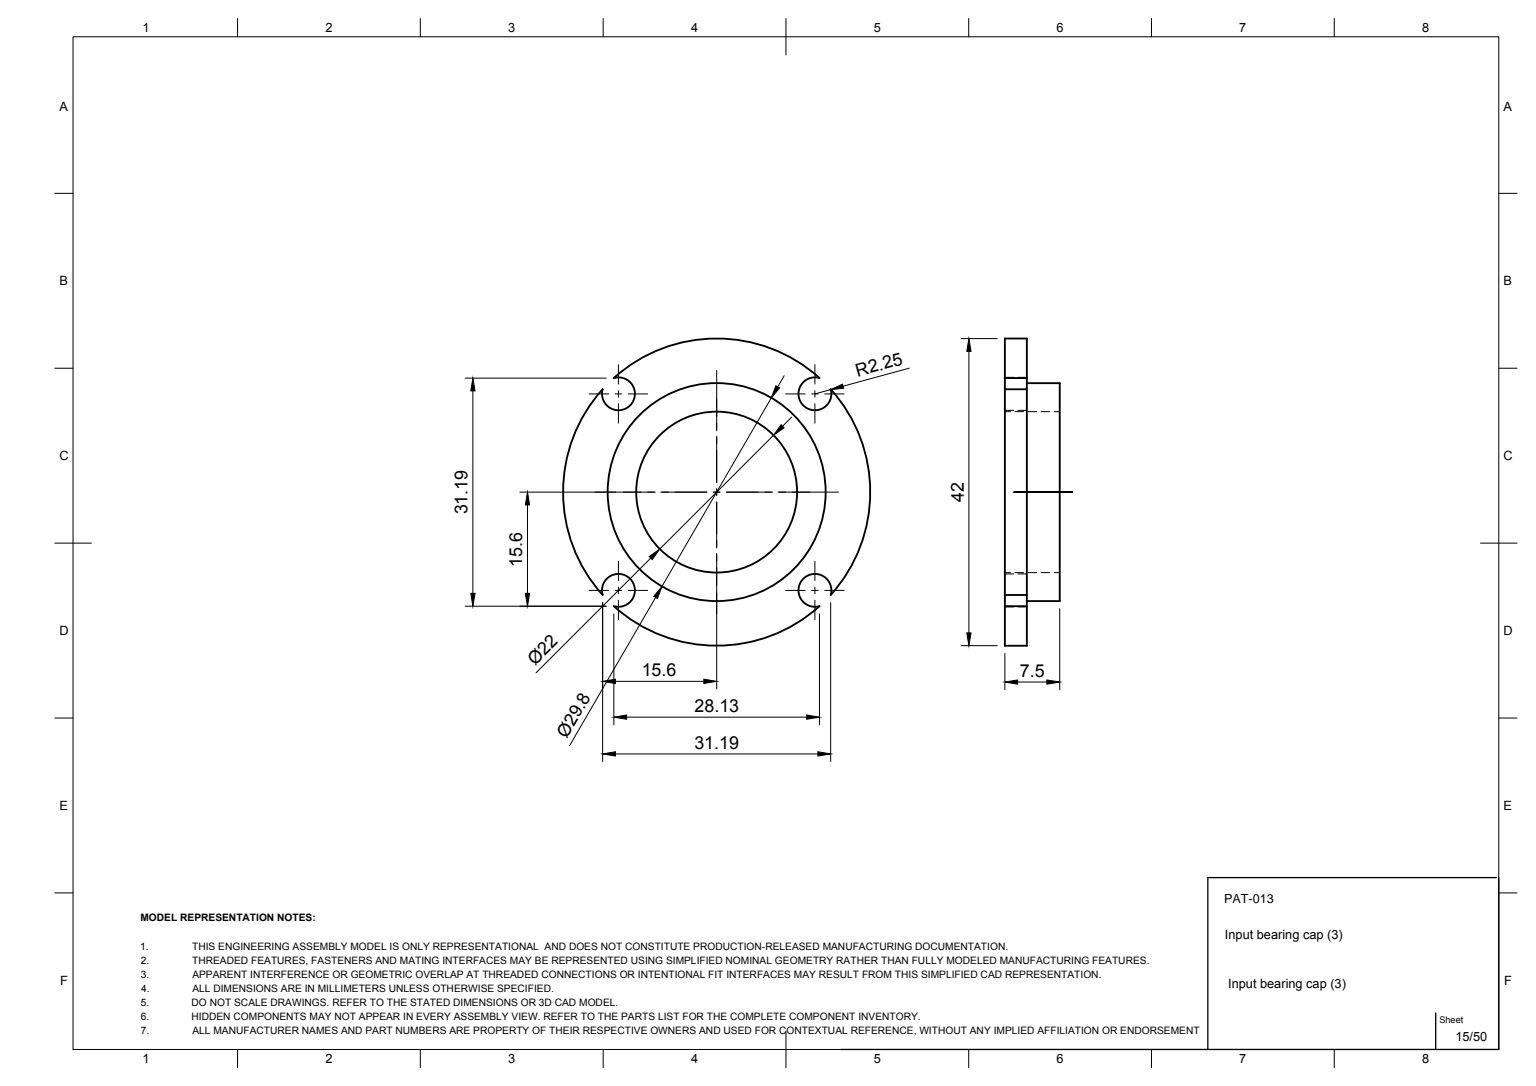
ISO-10303-21;
HEADER;
/* Generated by software containing ST-Developer
 * from STEP Tools, Inc. (www.steptools.com) 
 */

FILE_DESCRIPTION(
/* description */ ('Belt-driven linear axis on 2020 extrusion'),
/* implementation_level */ '2;1');

FILE_NAME(
/* name */ 'Input bearing cap (3).step',
/* time_stamp */ '2026-10-28T03:26:09-07:00',
/* author */ (''),
/* organization */ (''),
/* preprocessor_version */ 'ST-DEVELOPER v20.2',
/* originating_system */ 'Autodesk Translation Framework v15.17.0.0',
/* authorisation */ '');

FILE_SCHEMA (('AUTOMOTIVE_DESIGN { 1 0 10303 214 3 1 1 }'));
ENDSEC;

DATA;
#10=MECHANICAL_DESIGN_GEOMETRIC_PRESENTATION_REPRESENTATION('',(#622),#20096);
#528=SHAPE_REPRESENTATION_RELATIONSHIP('SRR','None',#20324,#574);
#574=ADVANCED_BREP_SHAPE_REPRESENTATION('',(#678),#20055);
#622=STYLED_ITEM('',(#20650),#678);
#678=MANIFOLD_SOLID_BREP('Body1',#10935);
#791=FACE_BOUND('',#2101,.T.);
#792=FACE_BOUND('',#2108,.T.);
#793=FACE_BOUND('',#2111,.T.);
#968=PLANE('',#11810);
#969=PLANE('',#11826);
#970=PLANE('',#11830);
#1401=FACE_OUTER_BOUND('',#2096,.T.);
#1402=FACE_OUTER_BOUND('',#2097,.T.);
#1403=FACE_OUTER_BOUND('',#2098,.T.);
#1404=FACE_OUTER_BOUND('',#2099,.T.);
#1405=FACE_OUTER_BOUND('',#2100,.T.);
#1406=FACE_OUTER_BOUND('',#2102,.T.);
#1407=FACE_OUTER_BOUND('',#2103,.T.);
#1408=FACE_OUTER_BOUND('',#2104,.T.);
#1409=FACE_OUTER_BOUND('',#2105,.T.);
#1410=FACE_OUTER_BOUND('',#2106,.T.);
#1411=FACE_OUTER_BOUND('',#2107,.T.);
#1412=FACE_OUTER_BOUND('',#2109,.T.);
#1413=FACE_OUTER_BOUND('',#2110,.T.);
#2096=EDGE_LOOP('',(#7901,#7902,#7903,#7904));
#2097=EDGE_LOOP('',(#7905,#7906,#7907,#7908));
#2098=EDGE_LOOP('',(#7909,#7910,#7911,#7912));
#2099=EDGE_LOOP('',(#7913,#7914,#7915,#7916));
#2100=EDGE_LOOP('',(#7917,#7918,#7919,#7920,#7921,#7922,#7923,#7924));
#2101=EDGE_LOOP('',(#7925));
#2102=EDGE_LOOP('',(#7926,#7927,#7928,#7929));
#2103=EDGE_LOOP('',(#7930,#7931,#7932,#7933));
#2104=EDGE_LOOP('',(#7934,#7935,#7936,#7937));
#2105=EDGE_LOOP('',(#7938,#7939,#7940,#7941));
#2106=EDGE_LOOP('',(#7942,#7943,#7944,#7945));
#2107=EDGE_LOOP('',(#7946));
#2108=EDGE_LOOP('',(#7947));
#2109=EDGE_LOOP('',(#7948,#7949,#7950,#7951));
#2110=EDGE_LOOP('',(#7952,#7953,#7954,#7955,#7956,#7957,#7958,#7959));
#2111=EDGE_LOOP('',(#7960));
#2845=LINE('',#16939,#3702);
#2846=LINE('',#16943,#3703);
#2847=LINE('',#16948,#3704);
#2848=LINE('',#16952,#3705);
#2849=LINE('',#16957,#3706);
#2850=LINE('',#16961,#3707);
#2851=LINE('',#16966,#3708);
#2852=LINE('',#16970,#3709);
#2853=LINE('',#16989,#3710);
#2854=LINE('',#16997,#3711);
#3702=VECTOR('',#13583,1.);
#3703=VECTOR('',#13586,1.);
#3704=VECTOR('',#13591,1.);
#3705=VECTOR('',#13594,1.);
#3706=VECTOR('',#13599,1.);
#3707=VECTOR('',#13602,1.);
#3708=VECTOR('',#13607,1.);
#3709=VECTOR('',#13610,1.);
#3710=VECTOR('',#13643,1.49);
#3711=VECTOR('',#13654,1.1);
#4523=CIRCLE('',#11799,0.225000000000001);
#4524=CIRCLE('',#11800,0.225000000000001);
#4525=CIRCLE('',#11802,0.225000000000001);
#4526=CIRCLE('',#11803,0.225000000000001);
#4527=CIRCLE('',#11805,0.225000000000001);
#4528=CIRCLE('',#11806,0.225000000000001);
#4529=CIRCLE('',#11808,0.225000000000001);
#4530=CIRCLE('',#11809,0.225000000000001);
#4531=CIRCLE('',#11811,2.1);
#4532=CIRCLE('',#11812,2.1);
#4533=CIRCLE('',#11813,2.1);
#4534=CIRCLE('',#11814,2.1);
#4535=CIRCLE('',#11815,1.49);
#4536=CIRCLE('',#11817,2.1);
#4537=CIRCLE('',#11819,2.1);
#4538=CIRCLE('',#11821,2.1);
#4539=CIRCLE('',#11823,2.1);
#4540=CIRCLE('',#11825,1.49);
#4541=CIRCLE('',#11827,1.1);
#4542=CIRCLE('',#11829,1.1);
#5108=VERTEX_POINT('',#16937);
#5109=VERTEX_POINT('',#16938);
#5110=VERTEX_POINT('',#16940);
#5111=VERTEX_POINT('',#16942);
#5112=VERTEX_POINT('',#16946);
#5113=VERTEX_POINT('',#16947);
#5114=VERTEX_POINT('',#16949);
#5115=VERTEX_POINT('',#16951);
#5116=VERTEX_POINT('',#16955);
#5117=VERTEX_POINT('',#16956);
#5118=VERTEX_POINT('',#16958);
#5119=VERTEX_POINT('',#16960);
#5120=VERTEX_POINT('',#16964);
#5121=VERTEX_POINT('',#16965);
#5122=VERTEX_POINT('',#16967);
#5123=VERTEX_POINT('',#16969);
#5124=VERTEX_POINT('',#16977);
#5125=VERTEX_POINT('',#16988);
#5126=VERTEX_POINT('',#16992);
#5127=VERTEX_POINT('',#16995);
#6165=EDGE_CURVE('',#5108,#5109,#2845,.T.);
#6166=EDGE_CURVE('',#5110,#5108,#4523,.T.);
#6167=EDGE_CURVE('',#5111,#5110,#2846,.T.);
#6168=EDGE_CURVE('',#5109,#5111,#4524,.T.);
#6169=EDGE_CURVE('',#5112,#5113,#2847,.T.);
#6170=EDGE_CURVE('',#5114,#5112,#4525,.T.);
#6171=EDGE_CURVE('',#5115,#5114,#2848,.T.);
#6172=EDGE_CURVE('',#5113,#5115,#4526,.T.);
#6173=EDGE_CURVE('',#5116,#5117,#2849,.T.);
#6174=EDGE_CURVE('',#5118,#5116,#4527,.T.);
#6175=EDGE_CURVE('',#5119,#5118,#2850,.T.);
#6176=EDGE_CURVE('',#5117,#5119,#4528,.T.);
#6177=EDGE_CURVE('',#5120,#5121,#2851,.T.);
#6178=EDGE_CURVE('',#5122,#5120,#4529,.T.);
#6179=EDGE_CURVE('',#5123,#5122,#2852,.T.);
#6180=EDGE_CURVE('',#5121,#5123,#4530,.T.);
#6181=EDGE_CURVE('',#5122,#5108,#4531,.T.);
#6182=EDGE_CURVE('',#5118,#5120,#4532,.T.);
#6183=EDGE_CURVE('',#5114,#5116,#4533,.T.);
#6184=EDGE_CURVE('',#5110,#5112,#4534,.T.);
#6185=EDGE_CURVE('',#5124,#5124,#4535,.T.);
#6186=EDGE_CURVE('',#5119,#5121,#4536,.T.);
#6187=EDGE_CURVE('',#5115,#5117,#4537,.T.);
#6188=EDGE_CURVE('',#5123,#5109,#4538,.T.);
#6189=EDGE_CURVE('',#5111,#5113,#4539,.T.);
#6190=EDGE_CURVE('',#5124,#5125,#2853,.T.);
#6191=EDGE_CURVE('',#5125,#5125,#4540,.T.);
#6192=EDGE_CURVE('',#5126,#5126,#4541,.T.);
#6193=EDGE_CURVE('',#5127,#5127,#4542,.T.);
#6194=EDGE_CURVE('',#5127,#5126,#2854,.T.);
#7901=ORIENTED_EDGE('',*,*,#6165,.F.);
#7902=ORIENTED_EDGE('',*,*,#6166,.F.);
#7903=ORIENTED_EDGE('',*,*,#6167,.F.);
#7904=ORIENTED_EDGE('',*,*,#6168,.F.);
#7905=ORIENTED_EDGE('',*,*,#6169,.F.);
#7906=ORIENTED_EDGE('',*,*,#6170,.F.);
#7907=ORIENTED_EDGE('',*,*,#6171,.F.);
#7908=ORIENTED_EDGE('',*,*,#6172,.F.);
#7909=ORIENTED_EDGE('',*,*,#6173,.F.);
#7910=ORIENTED_EDGE('',*,*,#6174,.F.);
#7911=ORIENTED_EDGE('',*,*,#6175,.F.);
#7912=ORIENTED_EDGE('',*,*,#6176,.F.);
#7913=ORIENTED_EDGE('',*,*,#6177,.F.);
#7914=ORIENTED_EDGE('',*,*,#6178,.F.);
#7915=ORIENTED_EDGE('',*,*,#6179,.F.);
#7916=ORIENTED_EDGE('',*,*,#6180,.F.);
#7917=ORIENTED_EDGE('',*,*,#6166,.T.);
#7918=ORIENTED_EDGE('',*,*,#6181,.F.);
#7919=ORIENTED_EDGE('',*,*,#6178,.T.);
#7920=ORIENTED_EDGE('',*,*,#6182,.F.);
#7921=ORIENTED_EDGE('',*,*,#6174,.T.);
#7922=ORIENTED_EDGE('',*,*,#6183,.F.);
#7923=ORIENTED_EDGE('',*,*,#6170,.T.);
#7924=ORIENTED_EDGE('',*,*,#6184,.F.);
#7925=ORIENTED_EDGE('',*,*,#6185,.T.);
#7926=ORIENTED_EDGE('',*,*,#6175,.T.);
#7927=ORIENTED_EDGE('',*,*,#6182,.T.);
#7928=ORIENTED_EDGE('',*,*,#6177,.T.);
#7929=ORIENTED_EDGE('',*,*,#6186,.F.);
#7930=ORIENTED_EDGE('',*,*,#6171,.T.);
#7931=ORIENTED_EDGE('',*,*,#6183,.T.);
#7932=ORIENTED_EDGE('',*,*,#6173,.T.);
#7933=ORIENTED_EDGE('',*,*,#6187,.F.);
#7934=ORIENTED_EDGE('',*,*,#6165,.T.);
#7935=ORIENTED_EDGE('',*,*,#6188,.F.);
#7936=ORIENTED_EDGE('',*,*,#6179,.T.);
#7937=ORIENTED_EDGE('',*,*,#6181,.T.);
#7938=ORIENTED_EDGE('',*,*,#6167,.T.);
#7939=ORIENTED_EDGE('',*,*,#6184,.T.);
#7940=ORIENTED_EDGE('',*,*,#6169,.T.);
#7941=ORIENTED_EDGE('',*,*,#6189,.F.);
#7942=ORIENTED_EDGE('',*,*,#6185,.F.);
#7943=ORIENTED_EDGE('',*,*,#6190,.T.);
#7944=ORIENTED_EDGE('',*,*,#6191,.T.);
#7945=ORIENTED_EDGE('',*,*,#6190,.F.);
#7946=ORIENTED_EDGE('',*,*,#6191,.F.);
#7947=ORIENTED_EDGE('',*,*,#6192,.F.);
#7948=ORIENTED_EDGE('',*,*,#6193,.F.);
#7949=ORIENTED_EDGE('',*,*,#6194,.T.);
#7950=ORIENTED_EDGE('',*,*,#6192,.T.);
#7951=ORIENTED_EDGE('',*,*,#6194,.F.);
#7952=ORIENTED_EDGE('',*,*,#6168,.T.);
#7953=ORIENTED_EDGE('',*,*,#6189,.T.);
#7954=ORIENTED_EDGE('',*,*,#6172,.T.);
#7955=ORIENTED_EDGE('',*,*,#6187,.T.);
#7956=ORIENTED_EDGE('',*,*,#6176,.T.);
#7957=ORIENTED_EDGE('',*,*,#6186,.T.);
#7958=ORIENTED_EDGE('',*,*,#6180,.T.);
#7959=ORIENTED_EDGE('',*,*,#6188,.T.);
#7960=ORIENTED_EDGE('',*,*,#6193,.T.);
#10149=CYLINDRICAL_SURFACE('',#11798,0.225000000000001);
#10150=CYLINDRICAL_SURFACE('',#11801,0.225000000000001);
#10151=CYLINDRICAL_SURFACE('',#11804,0.225000000000001);
#10152=CYLINDRICAL_SURFACE('',#11807,0.225000000000001);
#10153=CYLINDRICAL_SURFACE('',#11816,2.1);
#10154=CYLINDRICAL_SURFACE('',#11818,2.1);
#10155=CYLINDRICAL_SURFACE('',#11820,2.1);
#10156=CYLINDRICAL_SURFACE('',#11822,2.1);
#10157=CYLINDRICAL_SURFACE('',#11824,1.49);
#10158=CYLINDRICAL_SURFACE('',#11828,1.1);
#10452=ADVANCED_FACE('',(#1401),#10149,.F.);
#10453=ADVANCED_FACE('',(#1402),#10150,.F.);
#10454=ADVANCED_FACE('',(#1403),#10151,.F.);
#10455=ADVANCED_FACE('',(#1404),#10152,.F.);
#10456=ADVANCED_FACE('',(#1405,#791),#968,.F.);
#10457=ADVANCED_FACE('',(#1406),#10153,.T.);
#10458=ADVANCED_FACE('',(#1407),#10154,.T.);
#10459=ADVANCED_FACE('',(#1408),#10155,.T.);
#10460=ADVANCED_FACE('',(#1409),#10156,.T.);
#10461=ADVANCED_FACE('',(#1410),#10157,.T.);
#10462=ADVANCED_FACE('',(#1411,#792),#969,.F.);
#10463=ADVANCED_FACE('',(#1412),#10158,.F.);
#10464=ADVANCED_FACE('',(#1413,#793),#970,.T.);
#10935=CLOSED_SHELL('',(#10452,#10453,#10454,#10455,#10456,#10457,#10458,
#10459,#10460,#10461,#10462,#10463,#10464));
#11797=AXIS2_PLACEMENT_3D('',#16935,#13579,#13580);
#11798=AXIS2_PLACEMENT_3D('',#16936,#13581,#13582);
#11799=AXIS2_PLACEMENT_3D('',#16941,#13584,#13585);
#11800=AXIS2_PLACEMENT_3D('',#16944,#13587,#13588);
#11801=AXIS2_PLACEMENT_3D('',#16945,#13589,#13590);
#11802=AXIS2_PLACEMENT_3D('',#16950,#13592,#13593);
#11803=AXIS2_PLACEMENT_3D('',#16953,#13595,#13596);
#11804=AXIS2_PLACEMENT_3D('',#16954,#13597,#13598);
#11805=AXIS2_PLACEMENT_3D('',#16959,#13600,#13601);
#11806=AXIS2_PLACEMENT_3D('',#16962,#13603,#13604);
#11807=AXIS2_PLACEMENT_3D('',#16963,#13605,#13606);
#11808=AXIS2_PLACEMENT_3D('',#16968,#13608,#13609);
#11809=AXIS2_PLACEMENT_3D('',#16971,#13611,#13612);
#11810=AXIS2_PLACEMENT_3D('',#16972,#13613,#13614);
#11811=AXIS2_PLACEMENT_3D('',#16973,#13615,#13616);
#11812=AXIS2_PLACEMENT_3D('',#16974,#13617,#13618);
#11813=AXIS2_PLACEMENT_3D('',#16975,#13619,#13620);
#11814=AXIS2_PLACEMENT_3D('',#16976,#13621,#13622);
#11815=AXIS2_PLACEMENT_3D('',#16978,#13623,#13624);
#11816=AXIS2_PLACEMENT_3D('',#16979,#13625,#13626);
#11817=AXIS2_PLACEMENT_3D('',#16980,#13627,#13628);
#11818=AXIS2_PLACEMENT_3D('',#16981,#13629,#13630);
#11819=AXIS2_PLACEMENT_3D('',#16982,#13631,#13632);
#11820=AXIS2_PLACEMENT_3D('',#16983,#13633,#13634);
#11821=AXIS2_PLACEMENT_3D('',#16984,#13635,#13636);
#11822=AXIS2_PLACEMENT_3D('',#16985,#13637,#13638);
#11823=AXIS2_PLACEMENT_3D('',#16986,#13639,#13640);
#11824=AXIS2_PLACEMENT_3D('',#16987,#13641,#13642);
#11825=AXIS2_PLACEMENT_3D('',#16990,#13644,#13645);
#11826=AXIS2_PLACEMENT_3D('',#16991,#13646,#13647);
#11827=AXIS2_PLACEMENT_3D('',#16993,#13648,#13649);
#11828=AXIS2_PLACEMENT_3D('',#16994,#13650,#13651);
#11829=AXIS2_PLACEMENT_3D('',#16996,#13652,#13653);
#11830=AXIS2_PLACEMENT_3D('',#16998,#13655,#13656);
#13579=DIRECTION('axis',(0.,0.,1.));
#13580=DIRECTION('refdir',(1.,0.,0.));
#13581=DIRECTION('center_axis',(0.,1.,0.));
#13582=DIRECTION('ref_axis',(0.70710678118656,0.,0.707106781186535));
#13583=DIRECTION('',(0.,1.,0.));
#13584=DIRECTION('center_axis',(0.,1.,0.));
#13585=DIRECTION('ref_axis',(1.,0.,0.));
#13586=DIRECTION('',(0.,-1.,0.));
#13587=DIRECTION('center_axis',(0.,-1.,0.));
#13588=DIRECTION('ref_axis',(1.,0.,0.));
#13589=DIRECTION('center_axis',(0.,1.,0.));
#13590=DIRECTION('ref_axis',(0.707106781186561,0.,-0.707106781186534));
#13591=DIRECTION('',(0.,1.,0.));
#13592=DIRECTION('center_axis',(0.,1.,0.));
#13593=DIRECTION('ref_axis',(1.,0.,0.));
#13594=DIRECTION('',(0.,-1.,0.));
#13595=DIRECTION('center_axis',(0.,-1.,0.));
#13596=DIRECTION('ref_axis',(1.,0.,0.));
#13597=DIRECTION('center_axis',(0.,1.,0.));
#13598=DIRECTION('ref_axis',(-0.707106781186554,0.,-0.707106781186541));
#13599=DIRECTION('',(0.,1.,0.));
#13600=DIRECTION('center_axis',(0.,1.,0.));
#13601=DIRECTION('ref_axis',(1.,0.,0.));
#13602=DIRECTION('',(0.,-1.,0.));
#13603=DIRECTION('center_axis',(0.,-1.,0.));
#13604=DIRECTION('ref_axis',(1.,0.,0.));
#13605=DIRECTION('center_axis',(0.,1.,0.));
#13606=DIRECTION('ref_axis',(-0.707106781186554,0.,0.707106781186541));
#13607=DIRECTION('',(0.,1.,0.));
#13608=DIRECTION('center_axis',(0.,1.,0.));
#13609=DIRECTION('ref_axis',(1.,0.,0.));
#13610=DIRECTION('',(0.,-1.,0.));
#13611=DIRECTION('center_axis',(0.,-1.,0.));
#13612=DIRECTION('ref_axis',(1.,0.,0.));
#13613=DIRECTION('center_axis',(0.,1.,0.));
#13614=DIRECTION('ref_axis',(1.,0.,0.));
#13615=DIRECTION('center_axis',(0.,1.,0.));
#13616=DIRECTION('ref_axis',(1.,0.,0.));
#13617=DIRECTION('center_axis',(0.,1.,0.));
#13618=DIRECTION('ref_axis',(1.,0.,0.));
#13619=DIRECTION('center_axis',(0.,1.,0.));
#13620=DIRECTION('ref_axis',(1.,0.,0.));
#13621=DIRECTION('center_axis',(0.,1.,0.));
#13622=DIRECTION('ref_axis',(1.,0.,0.));
#13623=DIRECTION('center_axis',(0.,1.,0.));
#13624=DIRECTION('ref_axis',(1.,0.,0.));
#13625=DIRECTION('center_axis',(0.,1.,0.));
#13626=DIRECTION('ref_axis',(1.,0.,0.));
#13627=DIRECTION('center_axis',(0.,1.,0.));
#13628=DIRECTION('ref_axis',(1.,0.,0.));
#13629=DIRECTION('center_axis',(0.,1.,0.));
#13630=DIRECTION('ref_axis',(1.,0.,0.));
#13631=DIRECTION('center_axis',(0.,1.,0.));
#13632=DIRECTION('ref_axis',(1.,0.,0.));
#13633=DIRECTION('center_axis',(0.,1.,0.));
#13634=DIRECTION('ref_axis',(1.,0.,0.));
#13635=DIRECTION('center_axis',(0.,1.,0.));
#13636=DIRECTION('ref_axis',(1.,0.,0.));
#13637=DIRECTION('center_axis',(0.,1.,0.));
#13638=DIRECTION('ref_axis',(-1.,0.,-1.22464679914735E-16));
#13639=DIRECTION('center_axis',(0.,1.,0.));
#13640=DIRECTION('ref_axis',(1.,0.,0.));
#13641=DIRECTION('center_axis',(0.,1.,0.));
#13642=DIRECTION('ref_axis',(1.,0.,0.));
#13643=DIRECTION('',(0.,-1.,0.));
#13644=DIRECTION('center_axis',(0.,1.,0.));
#13645=DIRECTION('ref_axis',(1.,0.,0.));
#13646=DIRECTION('center_axis',(0.,1.,0.));
#13647=DIRECTION('ref_axis',(1.,0.,0.));
#13648=DIRECTION('center_axis',(0.,-1.,0.));
#13649=DIRECTION('ref_axis',(1.,0.,0.));
#13650=DIRECTION('center_axis',(0.,1.,0.));
#13651=DIRECTION('ref_axis',(1.,0.,0.));
#13652=DIRECTION('center_axis',(0.,-1.,0.));
#13653=DIRECTION('ref_axis',(1.,0.,0.));
#13654=DIRECTION('',(0.,-1.,0.));
#13655=DIRECTION('center_axis',(0.,1.,0.));
#13656=DIRECTION('ref_axis',(1.,0.,0.));
#16935=CARTESIAN_POINT('',(0.,0.,0.));
#16936=CARTESIAN_POINT('Origin',(30.6564971157456,1.7,5.65649711574556));
#16937=CARTESIAN_POINT('',(30.5936544441036,1.8,5.4404512904656));
#16938=CARTESIAN_POINT('',(30.5936544441036,2.1,5.4404512904656));
#16939=CARTESIAN_POINT('',(30.5936544441036,1.7,5.4404512904656));
#16940=CARTESIAN_POINT('',(30.4404512904656,1.8,5.59365444410359));
#16941=CARTESIAN_POINT('Origin',(30.6564971157456,1.8,5.65649711574556));
#16942=CARTESIAN_POINT('',(30.4404512904656,2.1,5.59365444410359));
#16943=CARTESIAN_POINT('',(30.4404512904656,1.7,5.59365444410359));
#16944=CARTESIAN_POINT('Origin',(30.6564971157456,2.1,5.65649711574556));
#16945=CARTESIAN_POINT('Origin',(30.6564971157456,1.7,8.34350288425444));
#16946=CARTESIAN_POINT('',(30.4404512904656,1.8,8.40634555589641));
#16947=CARTESIAN_POINT('',(30.4404512904656,2.1,8.40634555589641));
#16948=CARTESIAN_POINT('',(30.4404512904656,1.7,8.40634555589641));
#16949=CARTESIAN_POINT('',(30.5936544441036,1.8,8.5595487095344));
#16950=CARTESIAN_POINT('Origin',(30.6564971157456,1.8,8.34350288425444));
#16951=CARTESIAN_POINT('',(30.5936544441036,2.1,8.5595487095344));
#16952=CARTESIAN_POINT('',(30.5936544441036,1.7,8.5595487095344));
#16953=CARTESIAN_POINT('Origin',(30.6564971157456,2.1,8.34350288425444));
#16954=CARTESIAN_POINT('Origin',(33.3435028842544,1.7,8.34350288425444));
#16955=CARTESIAN_POINT('',(33.4063455558964,1.8,8.5595487095344));
#16956=CARTESIAN_POINT('',(33.4063455558964,2.1,8.5595487095344));
#16957=CARTESIAN_POINT('',(33.4063455558964,1.7,8.5595487095344));
#16958=CARTESIAN_POINT('',(33.5595487095344,1.8,8.40634555589641));
#16959=CARTESIAN_POINT('Origin',(33.3435028842544,1.8,8.34350288425444));
#16960=CARTESIAN_POINT('',(33.5595487095344,2.1,8.40634555589641));
#16961=CARTESIAN_POINT('',(33.5595487095344,1.7,8.40634555589641));
#16962=CARTESIAN_POINT('Origin',(33.3435028842544,2.1,8.34350288425444));
#16963=CARTESIAN_POINT('Origin',(33.3435028842544,1.7,5.65649711574556));
#16964=CARTESIAN_POINT('',(33.5595487095344,1.8,5.59365444410359));
#16965=CARTESIAN_POINT('',(33.5595487095344,2.1,5.59365444410359));
#16966=CARTESIAN_POINT('',(33.5595487095344,1.7,5.59365444410359));
#16967=CARTESIAN_POINT('',(33.4063455558964,1.8,5.4404512904656));
#16968=CARTESIAN_POINT('Origin',(33.3435028842544,1.8,5.65649711574556));
#16969=CARTESIAN_POINT('',(33.4063455558964,2.1,5.4404512904656));
#16970=CARTESIAN_POINT('',(33.4063455558964,1.7,5.4404512904656));
#16971=CARTESIAN_POINT('Origin',(33.3435028842544,2.1,5.65649711574556));
#16972=CARTESIAN_POINT('Origin',(32.,1.8,7.));
#16973=CARTESIAN_POINT('Origin',(32.,1.8,7.));
#16974=CARTESIAN_POINT('Origin',(32.,1.8,7.));
#16975=CARTESIAN_POINT('Origin',(32.,1.8,7.));
#16976=CARTESIAN_POINT('Origin',(32.,1.8,7.));
#16977=CARTESIAN_POINT('',(30.51,1.8,7.));
#16978=CARTESIAN_POINT('Origin',(32.,1.8,7.));
#16979=CARTESIAN_POINT('Origin',(32.,1.8,7.));
#16980=CARTESIAN_POINT('Origin',(32.,2.1,7.));
#16981=CARTESIAN_POINT('Origin',(32.,1.8,7.));
#16982=CARTESIAN_POINT('Origin',(32.,2.1,7.));
#16983=CARTESIAN_POINT('Origin',(32.,1.8,7.));
#16984=CARTESIAN_POINT('Origin',(32.,2.1,7.));
#16985=CARTESIAN_POINT('Origin',(32.,1.8,7.));
#16986=CARTESIAN_POINT('Origin',(32.,2.1,7.));
#16987=CARTESIAN_POINT('Origin',(32.,1.35,7.));
#16988=CARTESIAN_POINT('',(30.51,1.35,7.));
#16989=CARTESIAN_POINT('',(30.51,1.35,7.));
#16990=CARTESIAN_POINT('Origin',(32.,1.35,7.));
#16991=CARTESIAN_POINT('Origin',(32.,1.35,7.));
#16992=CARTESIAN_POINT('',(30.9,1.35,7.));
#16993=CARTESIAN_POINT('Origin',(32.,1.35,7.));
#16994=CARTESIAN_POINT('Origin',(32.,1.8,7.));
#16995=CARTESIAN_POINT('',(30.9,2.1,7.));
#16996=CARTESIAN_POINT('Origin',(32.,2.1,7.));
#16997=CARTESIAN_POINT('',(30.9,1.8,7.));
#16998=CARTESIAN_POINT('Origin',(32.,2.1,7.));
#20001=UNCERTAINTY_MEASURE_WITH_UNIT(LENGTH_MEASURE(0.001),#20097,
'DISTANCE_ACCURACY_VALUE',
'Maximum model space distance between geometric entities at asserted c
onnectivities');
#20042=UNCERTAINTY_MEASURE_WITH_UNIT(LENGTH_MEASURE(0.001),#20097,
'DISTANCE_ACCURACY_VALUE',
'Maximum model space distance between geometric entities at asserted c
onnectivities');
#20055=(
GEOMETRIC_REPRESENTATION_CONTEXT(3)
GLOBAL_UNCERTAINTY_ASSIGNED_CONTEXT((#20001))
GLOBAL_UNIT_ASSIGNED_CONTEXT((#20097,#20099,#20100))
REPRESENTATION_CONTEXT('','3D')
);
#20096=(
GEOMETRIC_REPRESENTATION_CONTEXT(3)
GLOBAL_UNCERTAINTY_ASSIGNED_CONTEXT((#20042))
GLOBAL_UNIT_ASSIGNED_CONTEXT((#20097,#20099,#20100))
REPRESENTATION_CONTEXT('','3D')
);
#20097=(
LENGTH_UNIT()
NAMED_UNIT(*)
SI_UNIT(.CENTI.,.METRE.)
);
#20099=(
NAMED_UNIT(*)
PLANE_ANGLE_UNIT()
SI_UNIT($,.RADIAN.)
);
#20100=(
NAMED_UNIT(*)
SI_UNIT($,.STERADIAN.)
SOLID_ANGLE_UNIT()
);
#20113=SHAPE_DEFINITION_REPRESENTATION(#20166,#20324);
#20166=PRODUCT_DEFINITION_SHAPE('',$,#20378);
#20324=SHAPE_REPRESENTATION('',(#11797),#20055);
#20365=PRODUCT_DEFINITION_CONTEXT('part definition',#20526,'design');
#20378=PRODUCT_DEFINITION('Input bearing cap (3)','Input bearing cap (3)',
#20431,#20365);
#20431=PRODUCT_DEFINITION_FORMATION('',$,#20540);
#20526=APPLICATION_CONTEXT(
'Core Data for Automotive Mechanical Design Process');
#20527=PRODUCT_CONTEXT('part definition',#20526,'mechanical');
#20540=PRODUCT('Input bearing cap (3)','Input bearing cap (3)',
'Input bearing cap (3)',(#20527));
#20644=COLOUR_RGB('Grey',0.48,0.52,0.57);
#20645=FILL_AREA_STYLE_COLOUR('',#20644);
#20646=FILL_AREA_STYLE('',(#20645));
#20647=SURFACE_STYLE_FILL_AREA(#20646);
#20648=SURFACE_SIDE_STYLE('',(#20647));
#20649=SURFACE_STYLE_USAGE(.BOTH.,#20648);
#20650=PRESENTATION_STYLE_ASSIGNMENT((#20649));
ENDSEC;
END-ISO-10303-21;
